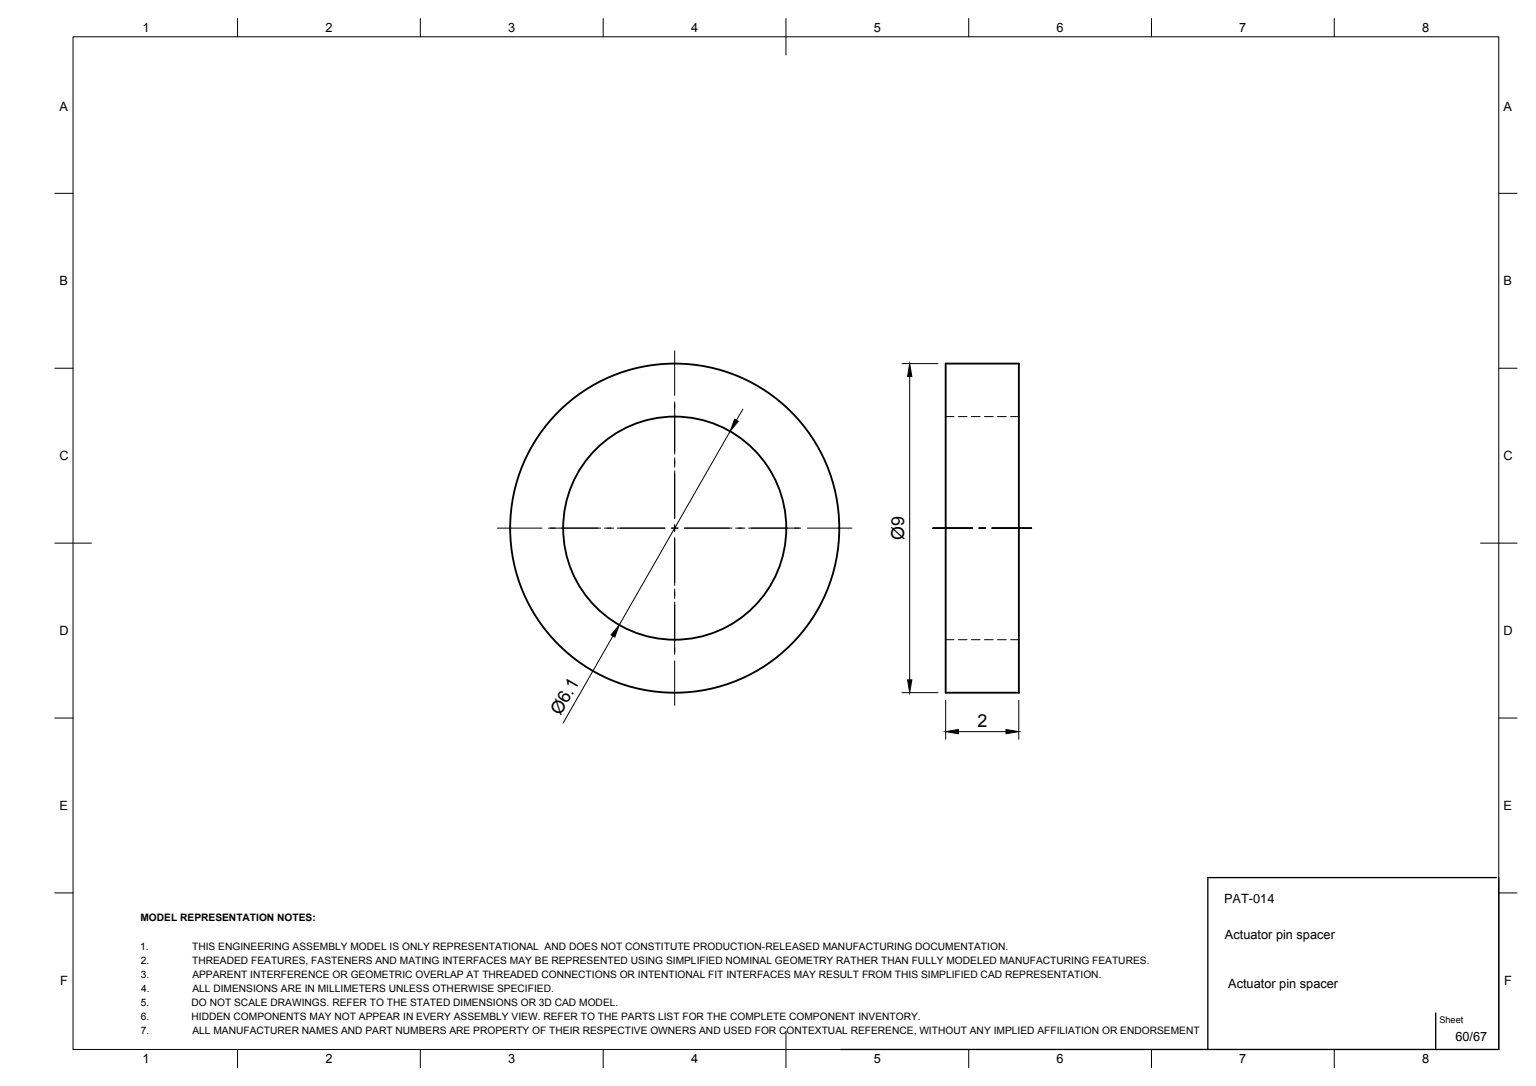
ISO-10303-21;
HEADER;
/* Generated by software containing ST-Developer
 * from STEP Tools, Inc. (www.steptools.com) 
 */

FILE_DESCRIPTION(
/* description */ ('Bin tilter linkage'),
/* implementation_level */ '2;1');

FILE_NAME(
/* name */ 'Actuator pin spacer.step',
/* time_stamp */ '2026-10-28T03:26:24-07:00',
/* author */ (''),
/* organization */ (''),
/* preprocessor_version */ 'ST-DEVELOPER v20.2',
/* originating_system */ 'Autodesk Translation Framework v15.17.0.0',
/* authorisation */ '');

FILE_SCHEMA (('AUTOMOTIVE_DESIGN { 1 0 10303 214 3 1 1 }'));
ENDSEC;

DATA;
#10=MECHANICAL_DESIGN_GEOMETRIC_PRESENTATION_REPRESENTATION('',(#966),#23728);
#746=SHAPE_REPRESENTATION_RELATIONSHIP('SRR','None',#24215,#852);
#852=ADVANCED_BREP_SHAPE_REPRESENTATION('',(#1078),#23715);
#966=STYLED_ITEM('',(#24765),#1078);
#1078=MANIFOLD_SOLID_BREP('Body1',#12498);
#1468=FACE_BOUND('',#3757,.T.);
#1469=FACE_BOUND('',#3759,.T.);
#1846=PLANE('',#15315);
#1847=PLANE('',#15316);
#2596=FACE_OUTER_BOUND('',#3754,.T.);
#2597=FACE_OUTER_BOUND('',#3755,.T.);
#2598=FACE_OUTER_BOUND('',#3756,.T.);
#2599=FACE_OUTER_BOUND('',#3758,.T.);
#3754=EDGE_LOOP('',(#11015,#11016,#11017,#11018));
#3755=EDGE_LOOP('',(#11019,#11020,#11021,#11022));
#3756=EDGE_LOOP('',(#11023));
#3757=EDGE_LOOP('',(#11024));
#3758=EDGE_LOOP('',(#11025));
#3759=EDGE_LOOP('',(#11026));
#4455=LINE('',#23182,#5130);
#4456=LINE('',#23188,#5131);
#5130=VECTOR('',#19350,0.305);
#5131=VECTOR('',#19357,0.45);
#5900=CIRCLE('',#15310,0.305);
#5901=CIRCLE('',#15311,0.305);
#5902=CIRCLE('',#15313,0.45);
#5903=CIRCLE('',#15314,0.45);
#6843=VERTEX_POINT('',#23179);
#6844=VERTEX_POINT('',#23181);
#6845=VERTEX_POINT('',#23185);
#6846=VERTEX_POINT('',#23187);
#8247=EDGE_CURVE('',#6843,#6843,#5900,.T.);
#8248=EDGE_CURVE('',#6843,#6844,#4455,.T.);
#8249=EDGE_CURVE('',#6844,#6844,#5901,.T.);
#8250=EDGE_CURVE('',#6845,#6845,#5902,.T.);
#8251=EDGE_CURVE('',#6845,#6846,#4456,.T.);
#8252=EDGE_CURVE('',#6846,#6846,#5903,.T.);
#11015=ORIENTED_EDGE('',*,*,#8247,.F.);
#11016=ORIENTED_EDGE('',*,*,#8248,.T.);
#11017=ORIENTED_EDGE('',*,*,#8249,.T.);
#11018=ORIENTED_EDGE('',*,*,#8248,.F.);
#11019=ORIENTED_EDGE('',*,*,#8250,.F.);
#11020=ORIENTED_EDGE('',*,*,#8251,.T.);
#11021=ORIENTED_EDGE('',*,*,#8252,.T.);
#11022=ORIENTED_EDGE('',*,*,#8251,.F.);
#11023=ORIENTED_EDGE('',*,*,#8250,.T.);
#11024=ORIENTED_EDGE('',*,*,#8247,.T.);
#11025=ORIENTED_EDGE('',*,*,#8252,.F.);
#11026=ORIENTED_EDGE('',*,*,#8249,.F.);
#11591=CYLINDRICAL_SURFACE('',#15309,0.305);
#11592=CYLINDRICAL_SURFACE('',#15312,0.45);
#12321=ADVANCED_FACE('',(#2596),#11591,.F.);
#12322=ADVANCED_FACE('',(#2597),#11592,.T.);
#12323=ADVANCED_FACE('',(#2598,#1468),#1846,.T.);
#12324=ADVANCED_FACE('',(#2599,#1469),#1847,.F.);
#12498=CLOSED_SHELL('',(#12321,#12322,#12323,#12324));
#15308=AXIS2_PLACEMENT_3D('',#23177,#19344,#19345);
#15309=AXIS2_PLACEMENT_3D('',#23178,#19346,#19347);
#15310=AXIS2_PLACEMENT_3D('',#23180,#19348,#19349);
#15311=AXIS2_PLACEMENT_3D('',#23183,#19351,#19352);
#15312=AXIS2_PLACEMENT_3D('',#23184,#19353,#19354);
#15313=AXIS2_PLACEMENT_3D('',#23186,#19355,#19356);
#15314=AXIS2_PLACEMENT_3D('',#23189,#19358,#19359);
#15315=AXIS2_PLACEMENT_3D('',#23190,#19360,#19361);
#15316=AXIS2_PLACEMENT_3D('',#23191,#19362,#19363);
#19344=DIRECTION('axis',(0.,0.,1.));
#19345=DIRECTION('refdir',(1.,0.,0.));
#19346=DIRECTION('center_axis',(0.,1.,0.));
#19347=DIRECTION('ref_axis',(1.,0.,0.));
#19348=DIRECTION('center_axis',(0.,-1.,0.));
#19349=DIRECTION('ref_axis',(1.,0.,0.));
#19350=DIRECTION('',(0.,-1.,0.));
#19351=DIRECTION('center_axis',(0.,-1.,0.));
#19352=DIRECTION('ref_axis',(1.,0.,0.));
#19353=DIRECTION('center_axis',(0.,1.,0.));
#19354=DIRECTION('ref_axis',(1.,0.,0.));
#19355=DIRECTION('center_axis',(0.,1.,0.));
#19356=DIRECTION('ref_axis',(1.,0.,0.));
#19357=DIRECTION('',(0.,-1.,0.));
#19358=DIRECTION('center_axis',(0.,1.,0.));
#19359=DIRECTION('ref_axis',(1.,0.,0.));
#19360=DIRECTION('center_axis',(0.,1.,0.));
#19361=DIRECTION('ref_axis',(1.,0.,0.));
#19362=DIRECTION('center_axis',(0.,1.,0.));
#19363=DIRECTION('ref_axis',(1.,0.,0.));
#23177=CARTESIAN_POINT('',(0.,0.,0.));
#23178=CARTESIAN_POINT('Origin',(-4.,-5.2,11.));
#23179=CARTESIAN_POINT('',(-4.305,-5.,11.));
#23180=CARTESIAN_POINT('Origin',(-4.,-5.,11.));
#23181=CARTESIAN_POINT('',(-4.305,-5.2,11.));
#23182=CARTESIAN_POINT('',(-4.305,-5.2,11.));
#23183=CARTESIAN_POINT('Origin',(-4.,-5.2,11.));
#23184=CARTESIAN_POINT('Origin',(-4.,-5.2,11.));
#23185=CARTESIAN_POINT('',(-4.45,-5.,11.));
#23186=CARTESIAN_POINT('Origin',(-4.,-5.,11.));
#23187=CARTESIAN_POINT('',(-4.45,-5.2,11.));
#23188=CARTESIAN_POINT('',(-4.45,-5.2,11.));
#23189=CARTESIAN_POINT('Origin',(-4.,-5.2,11.));
#23190=CARTESIAN_POINT('Origin',(-4.,-5.,11.));
#23191=CARTESIAN_POINT('Origin',(-4.,-5.2,11.));
#23598=UNCERTAINTY_MEASURE_WITH_UNIT(LENGTH_MEASURE(0.001),#23729,
'DISTANCE_ACCURACY_VALUE',
'Maximum model space distance between geometric entities at asserted c
onnectivities');
#23611=UNCERTAINTY_MEASURE_WITH_UNIT(LENGTH_MEASURE(0.001),#23729,
'DISTANCE_ACCURACY_VALUE',
'Maximum model space distance between geometric entities at asserted c
onnectivities');
#23715=(
GEOMETRIC_REPRESENTATION_CONTEXT(3)
GLOBAL_UNCERTAINTY_ASSIGNED_CONTEXT((#23598))
GLOBAL_UNIT_ASSIGNED_CONTEXT((#23729,#23731,#23732))
REPRESENTATION_CONTEXT('','3D')
);
#23728=(
GEOMETRIC_REPRESENTATION_CONTEXT(3)
GLOBAL_UNCERTAINTY_ASSIGNED_CONTEXT((#23611))
GLOBAL_UNIT_ASSIGNED_CONTEXT((#23729,#23731,#23732))
REPRESENTATION_CONTEXT('','3D')
);
#23729=(
LENGTH_UNIT()
NAMED_UNIT(*)
SI_UNIT(.CENTI.,.METRE.)
);
#23731=(
NAMED_UNIT(*)
PLANE_ANGLE_UNIT()
SI_UNIT($,.RADIAN.)
);
#23732=(
NAMED_UNIT(*)
SI_UNIT($,.STERADIAN.)
SOLID_ANGLE_UNIT()
);
#23836=SHAPE_DEFINITION_REPRESENTATION(#24074,#24215);
#24074=PRODUCT_DEFINITION_SHAPE('',$,#24332);
#24215=SHAPE_REPRESENTATION('',(#15308),#23715);
#24228=PRODUCT_DEFINITION_CONTEXT('part definition',#24578,'design');
#24332=PRODUCT_DEFINITION('Actuator pin spacer','Actuator pin spacer',#24448,
#24228);
#24448=PRODUCT_DEFINITION_FORMATION('',$,#24683);
#24578=APPLICATION_CONTEXT(
'Core Data for Automotive Mechanical Design Process');
#24579=PRODUCT_CONTEXT('part definition',#24578,'mechanical');
#24683=PRODUCT('Actuator pin spacer','Actuator pin spacer',
'Actuator pin spacer',(#24579));
#24759=COLOUR_RGB('Grey',0.48,0.52,0.57);
#24760=FILL_AREA_STYLE_COLOUR('',#24759);
#24761=FILL_AREA_STYLE('',(#24760));
#24762=SURFACE_STYLE_FILL_AREA(#24761);
#24763=SURFACE_SIDE_STYLE('',(#24762));
#24764=SURFACE_STYLE_USAGE(.BOTH.,#24763);
#24765=PRESENTATION_STYLE_ASSIGNMENT((#24764));
ENDSEC;
END-ISO-10303-21;
